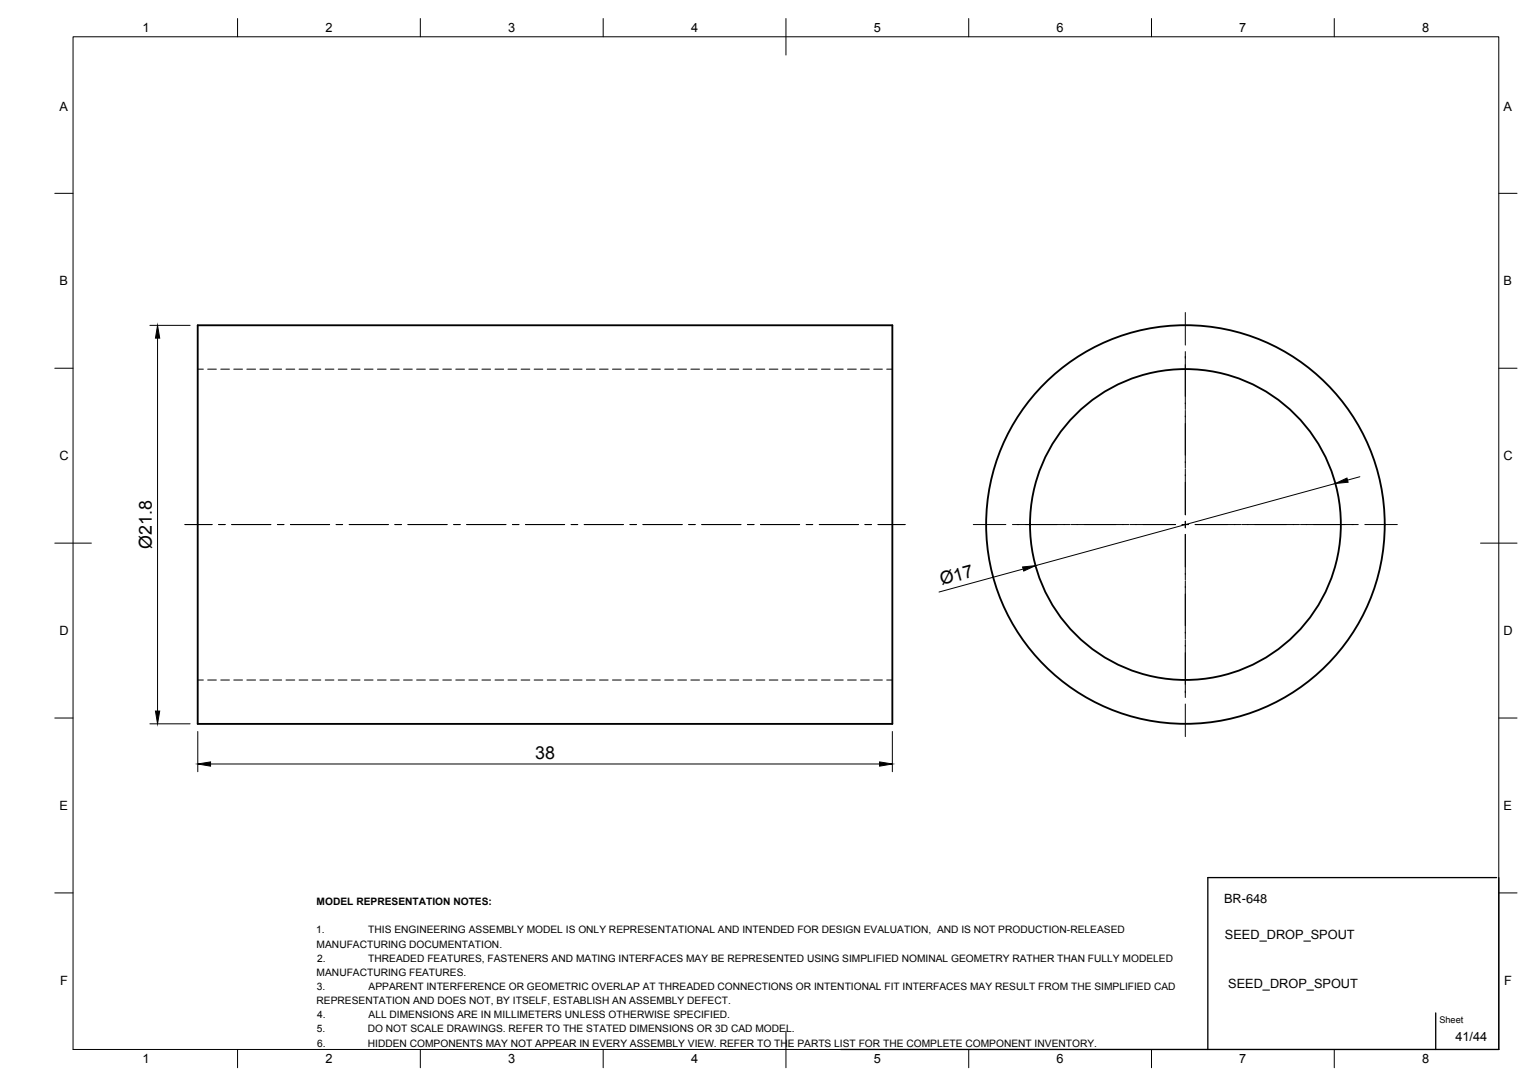
ISO-10303-21;
HEADER;
FILE_DESCRIPTION((''),'2;1');
FILE_NAME('SEED_DROP_SPOUT.step','2026-10-01T22:05:39-07:00',(''),(''),'','','');
FILE_SCHEMA (('AUTOMOTIVE_DESIGN { 1 0 10303 214 3 1 1 }'));
ENDSEC;
DATA;
#10=MECHANICAL_DESIGN_GEOMETRIC_PRESENTATION_REPRESENTATION('',(#637),#24628);
#553=SHAPE_REPRESENTATION_RELATIONSHIP('SRR','None',#24827,#595) ;
#595=ADVANCED_BREP_SHAPE_REPRESENTATION('',(#676),#24617) ;
#637=STYLED_ITEM('',(#25034),#676) ;
#676=MANIFOLD_SOLID_BREP('SEED_DROP_SPOUT',#13179) ;
#912=FACE_BOUND('',#4633,.T.) ;
#913=FACE_BOUND('',#4635,.T.) ;
#1722=LINE('',#24095,#2558) ;
#1723=LINE('',#24101,#2559) ;
#2558=VECTOR('',#19239,0.85) ;
#2559=VECTOR('',#19246,1.09) ;
#2924=CYLINDRICAL_SURFACE('',#15214,0.85) ;
#2925=CYLINDRICAL_SURFACE('',#15217,1.09) ;
#3637=FACE_OUTER_BOUND('',#4630,.T.) ;
#3638=FACE_OUTER_BOUND('',#4631,.T.) ;
#3639=FACE_OUTER_BOUND('',#4632,.T.) ;
#3640=FACE_OUTER_BOUND('',#4634,.T.) ;
#4630=EDGE_LOOP('',(#11653,#11654,#11655,#11656)) ;
#4631=EDGE_LOOP('',(#11657,#11658,#11659,#11660)) ;
#4632=EDGE_LOOP('',(#11661)) ;
#4633=EDGE_LOOP('',(#11662)) ;
#4634=EDGE_LOOP('',(#11663)) ;
#4635=EDGE_LOOP('',(#11664)) ;
#5483=CIRCLE('',#15215,0.85) ;
#5484=CIRCLE('',#15216,0.85) ;
#5485=CIRCLE('',#15218,1.09) ;
#5486=CIRCLE('',#15219,1.09) ;
#6619=VERTEX_POINT('',#24092) ;
#6620=VERTEX_POINT('',#24094) ;
#6621=VERTEX_POINT('',#24098) ;
#6622=VERTEX_POINT('',#24100) ;
#8316=EDGE_CURVE('',#6619,#6619,#5483,.T.) ;
#8317=EDGE_CURVE('',#6619,#6620,#1722,.T.) ;
#8318=EDGE_CURVE('',#6620,#6620,#5484,.T.) ;
#8319=EDGE_CURVE('',#6621,#6621,#5485,.T.) ;
#8320=EDGE_CURVE('',#6621,#6622,#1723,.T.) ;
#8321=EDGE_CURVE('',#6622,#6622,#5486,.T.) ;
#11653=ORIENTED_EDGE('',*,*,#8316,.F.) ;
#11654=ORIENTED_EDGE('',*,*,#8317,.T.) ;
#11655=ORIENTED_EDGE('',*,*,#8318,.F.) ;
#11656=ORIENTED_EDGE('',*,*,#8317,.F.) ;
#11657=ORIENTED_EDGE('',*,*,#8319,.F.) ;
#11658=ORIENTED_EDGE('',*,*,#8320,.T.) ;
#11659=ORIENTED_EDGE('',*,*,#8321,.F.) ;
#11660=ORIENTED_EDGE('',*,*,#8320,.F.) ;
#11661=ORIENTED_EDGE('',*,*,#8321,.T.) ;
#11662=ORIENTED_EDGE('',*,*,#8316,.T.) ;
#11663=ORIENTED_EDGE('',*,*,#8319,.T.) ;
#11664=ORIENTED_EDGE('',*,*,#8318,.T.) ;
#12293=PLANE('',#15220) ;
#12294=PLANE('',#15221) ;
#13032=ADVANCED_FACE('',(#3637),#2924,.F.) ;
#13033=ADVANCED_FACE('',(#3638),#2925,.T.) ;
#13034=ADVANCED_FACE('',(#3639,#912),#12293,.T.) ;
#13035=ADVANCED_FACE('',(#3640,#913),#12294,.T.) ;
#13179=CLOSED_SHELL('',(#13032,#13033,#13034,#13035)) ;
#15213=AXIS2_PLACEMENT_3D('',#24090,#19233,#19234) ;
#15214=AXIS2_PLACEMENT_3D('',#24091,#19235,#19236) ;
#15215=AXIS2_PLACEMENT_3D('',#24093,#19237,#19238) ;
#15216=AXIS2_PLACEMENT_3D('',#24096,#19240,#19241) ;
#15217=AXIS2_PLACEMENT_3D('',#24097,#19242,#19243) ;
#15218=AXIS2_PLACEMENT_3D('',#24099,#19244,#19245) ;
#15219=AXIS2_PLACEMENT_3D('',#24102,#19247,#19248) ;
#15220=AXIS2_PLACEMENT_3D('',#24103,#19249,#19250) ;
#15221=AXIS2_PLACEMENT_3D('',#24104,#19251,#19252) ;
#19233=DIRECTION('axis',(0.,0.,1.)) ;
#19234=DIRECTION('refdir',(1.,0.,0.)) ;
#19235=DIRECTION('center_axis',(0.,0.,1.)) ;
#19236=DIRECTION('ref_axis',(1.,0.,0.)) ;
#19237=DIRECTION('center_axis',(0.,0.,1.)) ;
#19238=DIRECTION('ref_axis',(1.,0.,0.)) ;
#19239=DIRECTION('',(0.,0.,1.)) ;
#19240=DIRECTION('center_axis',(0.,0.,-1.)) ;
#19241=DIRECTION('ref_axis',(1.,0.,0.)) ;
#19242=DIRECTION('center_axis',(0.,0.,1.)) ;
#19243=DIRECTION('ref_axis',(1.,0.,0.)) ;
#19244=DIRECTION('center_axis',(0.,0.,1.)) ;
#19245=DIRECTION('ref_axis',(1.,0.,0.)) ;
#19246=DIRECTION('',(0.,0.,-1.)) ;
#19247=DIRECTION('center_axis',(0.,0.,-1.)) ;
#19248=DIRECTION('ref_axis',(1.,0.,0.)) ;
#19249=DIRECTION('center_axis',(0.,0.,-1.)) ;
#19250=DIRECTION('ref_axis',(-1.,0.,0.)) ;
#19251=DIRECTION('center_axis',(0.,0.,1.)) ;
#19252=DIRECTION('ref_axis',(1.,0.,0.)) ;
#24090=CARTESIAN_POINT('',(0.,0.,0.)) ;
#24091=CARTESIAN_POINT('Origin',(-3.,-1.8,-13.2)) ;
#24092=CARTESIAN_POINT('',(-3.85,-1.8,-15.1)) ;
#24093=CARTESIAN_POINT('Origin',(-3.,-1.8,-15.1)) ;
#24094=CARTESIAN_POINT('',(-3.85,-1.8,-11.3)) ;
#24095=CARTESIAN_POINT('',(-3.85,-1.8,-13.2)) ;
#24096=CARTESIAN_POINT('Origin',(-3.,-1.8,-11.3)) ;
#24097=CARTESIAN_POINT('Origin',(-3.,-1.8,-13.2)) ;
#24098=CARTESIAN_POINT('',(-4.09,-1.8,-11.3)) ;
#24099=CARTESIAN_POINT('Origin',(-3.,-1.8,-11.3)) ;
#24100=CARTESIAN_POINT('',(-4.09,-1.8,-15.1)) ;
#24101=CARTESIAN_POINT('',(-4.09,-1.8,-13.2)) ;
#24102=CARTESIAN_POINT('Origin',(-3.,-1.8,-15.1)) ;
#24103=CARTESIAN_POINT('Origin',(-3.,-1.8,-15.1)) ;
#24104=CARTESIAN_POINT('Origin',(-3.,-1.8,-11.3)) ;
#24569=UNCERTAINTY_MEASURE_WITH_UNIT(LENGTH_MEASURE(0.001),#24629,
'DISTANCE_ACCURACY_VALUE',
'Maximum model space distance between geometric entities at asserted c
onnectivities') ;
#24580=UNCERTAINTY_MEASURE_WITH_UNIT(LENGTH_MEASURE(0.001),#24629,
'DISTANCE_ACCURACY_VALUE',
'Maximum model space distance between geometric entities at asserted c
onnectivities') ;
#24617=(
GEOMETRIC_REPRESENTATION_CONTEXT(3)
GLOBAL_UNCERTAINTY_ASSIGNED_CONTEXT((#24569))
GLOBAL_UNIT_ASSIGNED_CONTEXT((#24629,#24631,#24632))
REPRESENTATION_CONTEXT('','3D')
) ;
#24628=(
GEOMETRIC_REPRESENTATION_CONTEXT(3)
GLOBAL_UNCERTAINTY_ASSIGNED_CONTEXT((#24580))
GLOBAL_UNIT_ASSIGNED_CONTEXT((#24629,#24631,#24632))
REPRESENTATION_CONTEXT('','3D')
) ;
#24629=(
LENGTH_UNIT()
NAMED_UNIT(*)
SI_UNIT(.CENTI.,.METRE.)
) ;
#24631=(
NAMED_UNIT(*)
PLANE_ANGLE_UNIT()
SI_UNIT($,.RADIAN.)
) ;
#24632=(
NAMED_UNIT(*)
SI_UNIT($,.STERADIAN.)
SOLID_ANGLE_UNIT()
) ;
#24669=SHAPE_DEFINITION_REPRESENTATION(#24750,#24827) ;
#24750=PRODUCT_DEFINITION_SHAPE('',$,#24875) ;
#24827=SHAPE_REPRESENTATION('',(#15213),#24617) ;
#24838=PRODUCT_DEFINITION_CONTEXT('part definition',#24981,'design') ;
#24875=PRODUCT_DEFINITION('SEED_DROP_SPOUT','SEED_DROP_SPOUT',#24922,
#24838) ;
#24922=PRODUCT_DEFINITION_FORMATION('',$,#25019) ;
#24981=APPLICATION_CONTEXT(
'Core Data for Automotive Mechanical Design Process') ;
#24982=PRODUCT_CONTEXT('part definition',#24981,'mechanical') ;
#25019=PRODUCT('SEED_DROP_SPOUT','SEED_DROP_SPOUT',$,(#24982)) ;
#25034=PRESENTATION_STYLE_ASSIGNMENT((#25044)) ;
#25044=SURFACE_STYLE_USAGE(.BOTH.,#25054) ;
#25054=SURFACE_SIDE_STYLE('',(#25064)) ;
#25064=SURFACE_STYLE_FILL_AREA(#25074) ;
#25074=FILL_AREA_STYLE('Stainless Steel - Satin',(#25084)) ;
#25084=FILL_AREA_STYLE_COLOUR('Stainless Steel - Satin',#25094) ;
#25094=COLOUR_RGB('Stainless Steel - Satin', 0.31764706, 0.68627451, 0.89019608) ;
ENDSEC;
END-ISO-10303-21;
